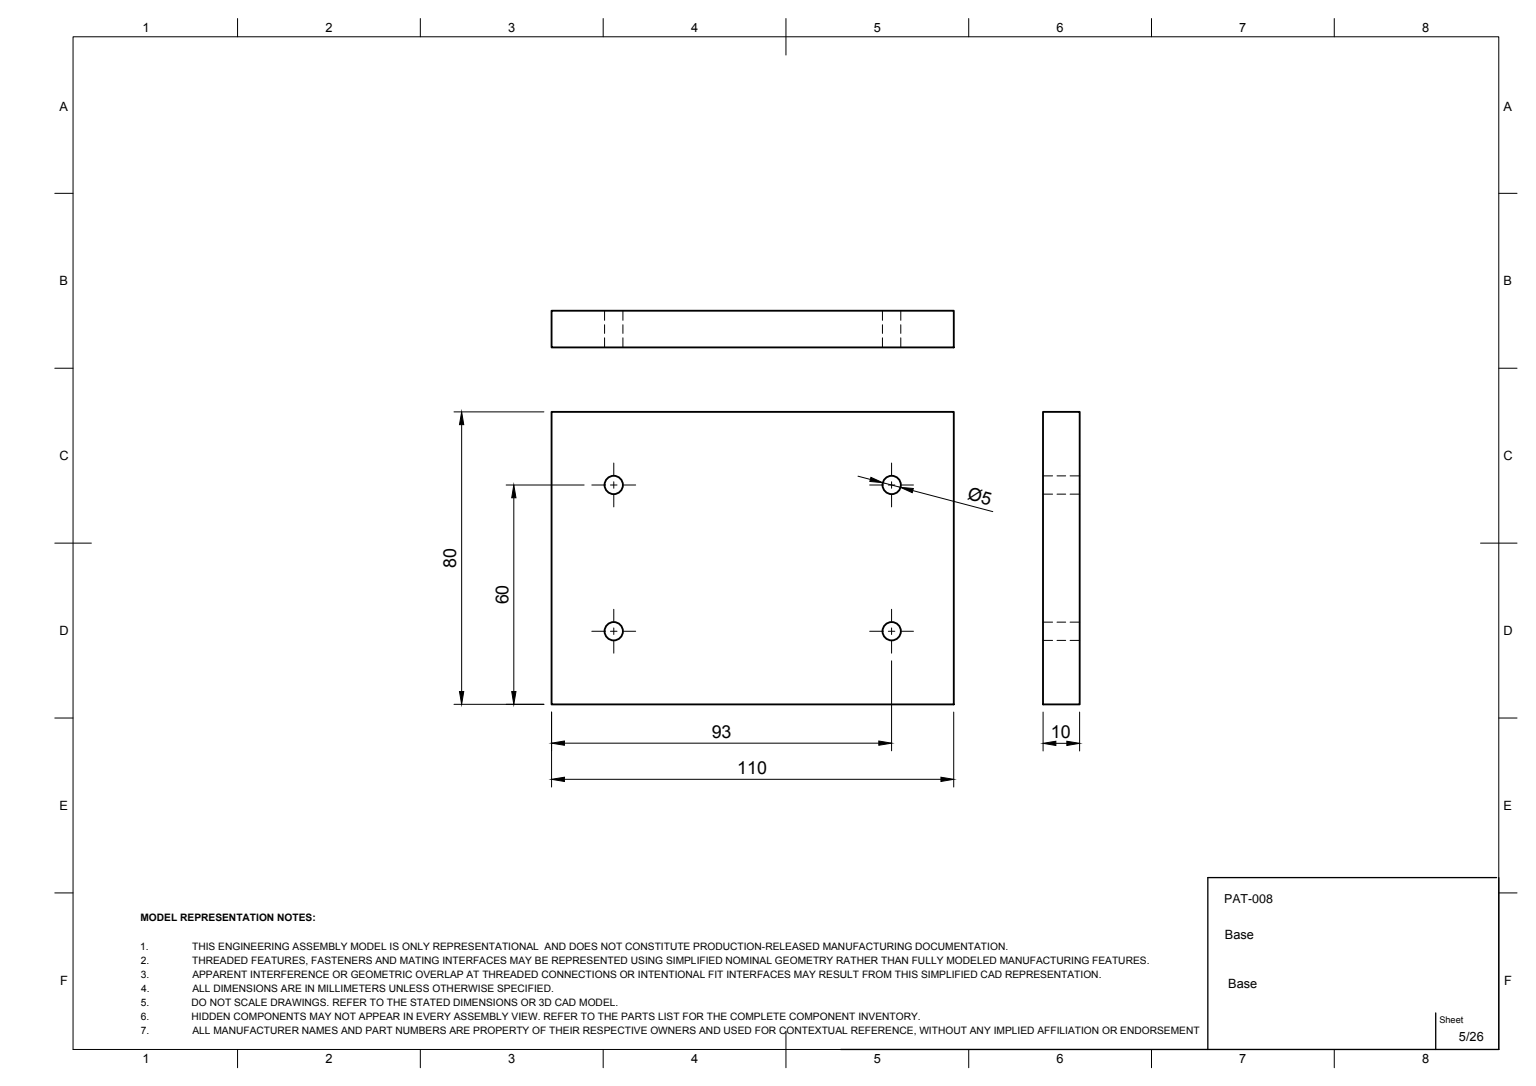
ISO-10303-21;
HEADER;
/* Generated by software containing ST-Developer
 * from STEP Tools, Inc. (www.steptools.com) 
 */

FILE_DESCRIPTION(
/* description */ ('Bearing housing with oil seal and end cap'),
/* implementation_level */ '2;1');

FILE_NAME(
/* name */ 'Base.step',
/* time_stamp */ '2026-10-28T03:23:10-07:00',
/* author */ (''),
/* organization */ (''),
/* preprocessor_version */ 'ST-DEVELOPER v20.2',
/* originating_system */ 'Autodesk Translation Framework v15.17.0.0',
/* authorisation */ '');

FILE_SCHEMA (('AUTOMOTIVE_DESIGN { 1 0 10303 214 3 1 1 }'));
ENDSEC;

DATA;
#10=MECHANICAL_DESIGN_GEOMETRIC_PRESENTATION_REPRESENTATION('',(#259),#7871);
#217=SHAPE_REPRESENTATION_RELATIONSHIP('SRR','None',#7964,#238);
#238=ADVANCED_BREP_SHAPE_REPRESENTATION('',(#288),#7848);
#259=STYLED_ITEM('',(#8132),#288);
#288=MANIFOLD_SOLID_BREP('Body1',#4085);
#315=FACE_BOUND('',#812,.T.);
#316=FACE_BOUND('',#813,.T.);
#317=FACE_BOUND('',#814,.T.);
#318=FACE_BOUND('',#815,.T.);
#319=FACE_BOUND('',#817,.T.);
#320=FACE_BOUND('',#818,.T.);
#321=FACE_BOUND('',#819,.T.);
#322=FACE_BOUND('',#820,.T.);
#408=PLANE('',#4363);
#409=PLANE('',#4364);
#410=PLANE('',#4365);
#411=PLANE('',#4366);
#412=PLANE('',#4367);
#413=PLANE('',#4368);
#552=FACE_OUTER_BOUND('',#803,.T.);
#553=FACE_OUTER_BOUND('',#804,.T.);
#554=FACE_OUTER_BOUND('',#805,.T.);
#555=FACE_OUTER_BOUND('',#806,.T.);
#556=FACE_OUTER_BOUND('',#807,.T.);
#557=FACE_OUTER_BOUND('',#808,.T.);
#558=FACE_OUTER_BOUND('',#809,.T.);
#559=FACE_OUTER_BOUND('',#810,.T.);
#560=FACE_OUTER_BOUND('',#811,.T.);
#561=FACE_OUTER_BOUND('',#816,.T.);
#803=EDGE_LOOP('',(#2743,#2744,#2745,#2746));
#804=EDGE_LOOP('',(#2747,#2748,#2749,#2750));
#805=EDGE_LOOP('',(#2751,#2752,#2753,#2754));
#806=EDGE_LOOP('',(#2755,#2756,#2757,#2758));
#807=EDGE_LOOP('',(#2759,#2760,#2761,#2762));
#808=EDGE_LOOP('',(#2763,#2764,#2765,#2766));
#809=EDGE_LOOP('',(#2767,#2768,#2769,#2770));
#810=EDGE_LOOP('',(#2771,#2772,#2773,#2774));
#811=EDGE_LOOP('',(#2775,#2776,#2777,#2778));
#812=EDGE_LOOP('',(#2779));
#813=EDGE_LOOP('',(#2780));
#814=EDGE_LOOP('',(#2781));
#815=EDGE_LOOP('',(#2782));
#816=EDGE_LOOP('',(#2783,#2784,#2785,#2786));
#817=EDGE_LOOP('',(#2787));
#818=EDGE_LOOP('',(#2788));
#819=EDGE_LOOP('',(#2789));
#820=EDGE_LOOP('',(#2790));
#1147=LINE('',#6213,#1409);
#1148=LINE('',#6219,#1410);
#1149=LINE('',#6225,#1411);
#1150=LINE('',#6231,#1412);
#1151=LINE('',#6236,#1413);
#1152=LINE('',#6238,#1414);
#1153=LINE('',#6240,#1415);
#1154=LINE('',#6241,#1416);
#1155=LINE('',#6244,#1417);
#1156=LINE('',#6246,#1418);
#1157=LINE('',#6247,#1419);
#1158=LINE('',#6250,#1420);
#1159=LINE('',#6252,#1421);
#1160=LINE('',#6253,#1422);
#1161=LINE('',#6255,#1423);
#1162=LINE('',#6256,#1424);
#1409=VECTOR('',#4890,0.25);
#1410=VECTOR('',#4897,0.25);
#1411=VECTOR('',#4904,0.25);
#1412=VECTOR('',#4911,0.25);
#1413=VECTOR('',#4916,1.);
#1414=VECTOR('',#4917,1.);
#1415=VECTOR('',#4918,1.);
#1416=VECTOR('',#4919,1.);
#1417=VECTOR('',#4922,1.);
#1418=VECTOR('',#4923,1.);
#1419=VECTOR('',#4924,1.);
#1420=VECTOR('',#4927,1.);
#1421=VECTOR('',#4928,1.);
#1422=VECTOR('',#4929,1.);
#1423=VECTOR('',#4932,1.);
#1424=VECTOR('',#4933,1.);
#1671=CIRCLE('',#4352,0.25);
#1672=CIRCLE('',#4353,0.25);
#1673=CIRCLE('',#4355,0.25);
#1674=CIRCLE('',#4356,0.25);
#1675=CIRCLE('',#4358,0.25);
#1676=CIRCLE('',#4359,0.25);
#1677=CIRCLE('',#4361,0.25);
#1678=CIRCLE('',#4362,0.25);
#1891=VERTEX_POINT('',#6210);
#1892=VERTEX_POINT('',#6212);
#1893=VERTEX_POINT('',#6216);
#1894=VERTEX_POINT('',#6218);
#1895=VERTEX_POINT('',#6222);
#1896=VERTEX_POINT('',#6224);
#1897=VERTEX_POINT('',#6228);
#1898=VERTEX_POINT('',#6230);
#1899=VERTEX_POINT('',#6234);
#1900=VERTEX_POINT('',#6235);
#1901=VERTEX_POINT('',#6237);
#1902=VERTEX_POINT('',#6239);
#1903=VERTEX_POINT('',#6243);
#1904=VERTEX_POINT('',#6245);
#1905=VERTEX_POINT('',#6249);
#1906=VERTEX_POINT('',#6251);
#2235=EDGE_CURVE('',#1891,#1891,#1671,.T.);
#2236=EDGE_CURVE('',#1891,#1892,#1147,.T.);
#2237=EDGE_CURVE('',#1892,#1892,#1672,.T.);
#2238=EDGE_CURVE('',#1893,#1893,#1673,.T.);
#2239=EDGE_CURVE('',#1893,#1894,#1148,.T.);
#2240=EDGE_CURVE('',#1894,#1894,#1674,.T.);
#2241=EDGE_CURVE('',#1895,#1895,#1675,.T.);
#2242=EDGE_CURVE('',#1895,#1896,#1149,.T.);
#2243=EDGE_CURVE('',#1896,#1896,#1676,.T.);
#2244=EDGE_CURVE('',#1897,#1897,#1677,.T.);
#2245=EDGE_CURVE('',#1897,#1898,#1150,.T.);
#2246=EDGE_CURVE('',#1898,#1898,#1678,.T.);
#2247=EDGE_CURVE('',#1899,#1900,#1151,.T.);
#2248=EDGE_CURVE('',#1900,#1901,#1152,.T.);
#2249=EDGE_CURVE('',#1902,#1901,#1153,.T.);
#2250=EDGE_CURVE('',#1899,#1902,#1154,.T.);
#2251=EDGE_CURVE('',#1903,#1899,#1155,.T.);
#2252=EDGE_CURVE('',#1904,#1902,#1156,.T.);
#2253=EDGE_CURVE('',#1903,#1904,#1157,.T.);
#2254=EDGE_CURVE('',#1905,#1903,#1158,.T.);
#2255=EDGE_CURVE('',#1906,#1904,#1159,.T.);
#2256=EDGE_CURVE('',#1905,#1906,#1160,.T.);
#2257=EDGE_CURVE('',#1900,#1905,#1161,.T.);
#2258=EDGE_CURVE('',#1901,#1906,#1162,.T.);
#2743=ORIENTED_EDGE('',*,*,#2235,.F.);
#2744=ORIENTED_EDGE('',*,*,#2236,.T.);
#2745=ORIENTED_EDGE('',*,*,#2237,.F.);
#2746=ORIENTED_EDGE('',*,*,#2236,.F.);
#2747=ORIENTED_EDGE('',*,*,#2238,.F.);
#2748=ORIENTED_EDGE('',*,*,#2239,.T.);
#2749=ORIENTED_EDGE('',*,*,#2240,.F.);
#2750=ORIENTED_EDGE('',*,*,#2239,.F.);
#2751=ORIENTED_EDGE('',*,*,#2241,.F.);
#2752=ORIENTED_EDGE('',*,*,#2242,.T.);
#2753=ORIENTED_EDGE('',*,*,#2243,.F.);
#2754=ORIENTED_EDGE('',*,*,#2242,.F.);
#2755=ORIENTED_EDGE('',*,*,#2244,.F.);
#2756=ORIENTED_EDGE('',*,*,#2245,.T.);
#2757=ORIENTED_EDGE('',*,*,#2246,.F.);
#2758=ORIENTED_EDGE('',*,*,#2245,.F.);
#2759=ORIENTED_EDGE('',*,*,#2247,.T.);
#2760=ORIENTED_EDGE('',*,*,#2248,.T.);
#2761=ORIENTED_EDGE('',*,*,#2249,.F.);
#2762=ORIENTED_EDGE('',*,*,#2250,.F.);
#2763=ORIENTED_EDGE('',*,*,#2251,.T.);
#2764=ORIENTED_EDGE('',*,*,#2250,.T.);
#2765=ORIENTED_EDGE('',*,*,#2252,.F.);
#2766=ORIENTED_EDGE('',*,*,#2253,.F.);
#2767=ORIENTED_EDGE('',*,*,#2254,.T.);
#2768=ORIENTED_EDGE('',*,*,#2253,.T.);
#2769=ORIENTED_EDGE('',*,*,#2255,.F.);
#2770=ORIENTED_EDGE('',*,*,#2256,.F.);
#2771=ORIENTED_EDGE('',*,*,#2257,.T.);
#2772=ORIENTED_EDGE('',*,*,#2256,.T.);
#2773=ORIENTED_EDGE('',*,*,#2258,.F.);
#2774=ORIENTED_EDGE('',*,*,#2248,.F.);
#2775=ORIENTED_EDGE('',*,*,#2258,.T.);
#2776=ORIENTED_EDGE('',*,*,#2255,.T.);
#2777=ORIENTED_EDGE('',*,*,#2252,.T.);
#2778=ORIENTED_EDGE('',*,*,#2249,.T.);
#2779=ORIENTED_EDGE('',*,*,#2237,.T.);
#2780=ORIENTED_EDGE('',*,*,#2240,.T.);
#2781=ORIENTED_EDGE('',*,*,#2243,.T.);
#2782=ORIENTED_EDGE('',*,*,#2246,.T.);
#2783=ORIENTED_EDGE('',*,*,#2257,.F.);
#2784=ORIENTED_EDGE('',*,*,#2247,.F.);
#2785=ORIENTED_EDGE('',*,*,#2251,.F.);
#2786=ORIENTED_EDGE('',*,*,#2254,.F.);
#2787=ORIENTED_EDGE('',*,*,#2235,.T.);
#2788=ORIENTED_EDGE('',*,*,#2238,.T.);
#2789=ORIENTED_EDGE('',*,*,#2241,.T.);
#2790=ORIENTED_EDGE('',*,*,#2244,.T.);
#3759=CYLINDRICAL_SURFACE('',#4351,0.25);
#3760=CYLINDRICAL_SURFACE('',#4354,0.25);
#3761=CYLINDRICAL_SURFACE('',#4357,0.25);
#3762=CYLINDRICAL_SURFACE('',#4360,0.25);
#3834=ADVANCED_FACE('',(#552),#3759,.F.);
#3835=ADVANCED_FACE('',(#553),#3760,.F.);
#3836=ADVANCED_FACE('',(#554),#3761,.F.);
#3837=ADVANCED_FACE('',(#555),#3762,.F.);
#3838=ADVANCED_FACE('',(#556),#408,.T.);
#3839=ADVANCED_FACE('',(#557),#409,.T.);
#3840=ADVANCED_FACE('',(#558),#410,.T.);
#3841=ADVANCED_FACE('',(#559),#411,.T.);
#3842=ADVANCED_FACE('',(#560,#315,#316,#317,#318),#412,.T.);
#3843=ADVANCED_FACE('',(#561,#319,#320,#321,#322),#413,.F.);
#4085=CLOSED_SHELL('',(#3834,#3835,#3836,#3837,#3838,#3839,#3840,#3841,
#3842,#3843));
#4350=AXIS2_PLACEMENT_3D('',#6208,#4884,#4885);
#4351=AXIS2_PLACEMENT_3D('',#6209,#4886,#4887);
#4352=AXIS2_PLACEMENT_3D('',#6211,#4888,#4889);
#4353=AXIS2_PLACEMENT_3D('',#6214,#4891,#4892);
#4354=AXIS2_PLACEMENT_3D('',#6215,#4893,#4894);
#4355=AXIS2_PLACEMENT_3D('',#6217,#4895,#4896);
#4356=AXIS2_PLACEMENT_3D('',#6220,#4898,#4899);
#4357=AXIS2_PLACEMENT_3D('',#6221,#4900,#4901);
#4358=AXIS2_PLACEMENT_3D('',#6223,#4902,#4903);
#4359=AXIS2_PLACEMENT_3D('',#6226,#4905,#4906);
#4360=AXIS2_PLACEMENT_3D('',#6227,#4907,#4908);
#4361=AXIS2_PLACEMENT_3D('',#6229,#4909,#4910);
#4362=AXIS2_PLACEMENT_3D('',#6232,#4912,#4913);
#4363=AXIS2_PLACEMENT_3D('',#6233,#4914,#4915);
#4364=AXIS2_PLACEMENT_3D('',#6242,#4920,#4921);
#4365=AXIS2_PLACEMENT_3D('',#6248,#4925,#4926);
#4366=AXIS2_PLACEMENT_3D('',#6254,#4930,#4931);
#4367=AXIS2_PLACEMENT_3D('',#6257,#4934,#4935);
#4368=AXIS2_PLACEMENT_3D('',#6258,#4936,#4937);
#4884=DIRECTION('axis',(0.,0.,1.));
#4885=DIRECTION('refdir',(1.,0.,0.));
#4886=DIRECTION('center_axis',(0.,0.,1.));
#4887=DIRECTION('ref_axis',(1.,0.,0.));
#4888=DIRECTION('center_axis',(0.,0.,1.));
#4889=DIRECTION('ref_axis',(1.,0.,0.));
#4890=DIRECTION('',(0.,0.,1.));
#4891=DIRECTION('center_axis',(0.,0.,-1.));
#4892=DIRECTION('ref_axis',(1.,0.,0.));
#4893=DIRECTION('center_axis',(0.,0.,1.));
#4894=DIRECTION('ref_axis',(1.,0.,0.));
#4895=DIRECTION('center_axis',(0.,0.,1.));
#4896=DIRECTION('ref_axis',(1.,0.,0.));
#4897=DIRECTION('',(0.,0.,1.));
#4898=DIRECTION('center_axis',(0.,0.,-1.));
#4899=DIRECTION('ref_axis',(1.,0.,0.));
#4900=DIRECTION('center_axis',(0.,0.,1.));
#4901=DIRECTION('ref_axis',(1.,0.,0.));
#4902=DIRECTION('center_axis',(0.,0.,1.));
#4903=DIRECTION('ref_axis',(1.,0.,0.));
#4904=DIRECTION('',(0.,0.,1.));
#4905=DIRECTION('center_axis',(0.,0.,-1.));
#4906=DIRECTION('ref_axis',(1.,0.,0.));
#4907=DIRECTION('center_axis',(0.,0.,1.));
#4908=DIRECTION('ref_axis',(1.,0.,0.));
#4909=DIRECTION('center_axis',(0.,0.,1.));
#4910=DIRECTION('ref_axis',(1.,0.,0.));
#4911=DIRECTION('',(0.,0.,1.));
#4912=DIRECTION('center_axis',(0.,0.,-1.));
#4913=DIRECTION('ref_axis',(1.,0.,0.));
#4914=DIRECTION('center_axis',(0.,1.,0.));
#4915=DIRECTION('ref_axis',(-1.,0.,0.));
#4916=DIRECTION('',(-1.,0.,0.));
#4917=DIRECTION('',(0.,0.,1.));
#4918=DIRECTION('',(-1.,0.,0.));
#4919=DIRECTION('',(0.,0.,1.));
#4920=DIRECTION('center_axis',(1.,0.,0.));
#4921=DIRECTION('ref_axis',(0.,1.,0.));
#4922=DIRECTION('',(0.,1.,0.));
#4923=DIRECTION('',(0.,1.,0.));
#4924=DIRECTION('',(0.,0.,1.));
#4925=DIRECTION('center_axis',(0.,-1.,0.));
#4926=DIRECTION('ref_axis',(1.,0.,0.));
#4927=DIRECTION('',(1.,0.,0.));
#4928=DIRECTION('',(1.,0.,0.));
#4929=DIRECTION('',(0.,0.,1.));
#4930=DIRECTION('center_axis',(-1.,0.,0.));
#4931=DIRECTION('ref_axis',(0.,-1.,0.));
#4932=DIRECTION('',(0.,-1.,0.));
#4933=DIRECTION('',(0.,-1.,0.));
#4934=DIRECTION('center_axis',(0.,0.,1.));
#4935=DIRECTION('ref_axis',(1.,0.,0.));
#4936=DIRECTION('center_axis',(0.,0.,1.));
#4937=DIRECTION('ref_axis',(1.,0.,0.));
#6208=CARTESIAN_POINT('',(0.,0.,0.));
#6209=CARTESIAN_POINT('Origin',(3.8,1.,-0.1));
#6210=CARTESIAN_POINT('',(3.55,1.,0.));
#6211=CARTESIAN_POINT('Origin',(3.8,1.,0.));
#6212=CARTESIAN_POINT('',(3.55,1.,1.));
#6213=CARTESIAN_POINT('',(3.55,1.,-0.1));
#6214=CARTESIAN_POINT('Origin',(3.8,1.,1.));
#6215=CARTESIAN_POINT('Origin',(-3.8,5.,-0.1));
#6216=CARTESIAN_POINT('',(-4.05,5.,0.));
#6217=CARTESIAN_POINT('Origin',(-3.8,5.,0.));
#6218=CARTESIAN_POINT('',(-4.05,5.,1.));
#6219=CARTESIAN_POINT('',(-4.05,5.,-0.1));
#6220=CARTESIAN_POINT('Origin',(-3.8,5.,1.));
#6221=CARTESIAN_POINT('Origin',(-3.8,1.,-0.1));
#6222=CARTESIAN_POINT('',(-4.05,1.,0.));
#6223=CARTESIAN_POINT('Origin',(-3.8,1.,0.));
#6224=CARTESIAN_POINT('',(-4.05,1.,1.));
#6225=CARTESIAN_POINT('',(-4.05,1.,-0.1));
#6226=CARTESIAN_POINT('Origin',(-3.8,1.,1.));
#6227=CARTESIAN_POINT('Origin',(3.8,5.,-0.1));
#6228=CARTESIAN_POINT('',(3.55,5.,0.));
#6229=CARTESIAN_POINT('Origin',(3.8,5.,0.));
#6230=CARTESIAN_POINT('',(3.55,5.,1.));
#6231=CARTESIAN_POINT('',(3.55,5.,-0.1));
#6232=CARTESIAN_POINT('Origin',(3.8,5.,1.));
#6233=CARTESIAN_POINT('Origin',(5.5,7.,0.));
#6234=CARTESIAN_POINT('',(5.5,7.,0.));
#6235=CARTESIAN_POINT('',(-5.5,7.,0.));
#6236=CARTESIAN_POINT('',(5.5,7.,0.));
#6237=CARTESIAN_POINT('',(-5.5,7.,1.));
#6238=CARTESIAN_POINT('',(-5.5,7.,0.));
#6239=CARTESIAN_POINT('',(5.5,7.,1.));
#6240=CARTESIAN_POINT('',(5.5,7.,1.));
#6241=CARTESIAN_POINT('',(5.5,7.,0.));
#6242=CARTESIAN_POINT('Origin',(5.5,-1.,0.));
#6243=CARTESIAN_POINT('',(5.5,-1.,0.));
#6244=CARTESIAN_POINT('',(5.5,-1.,0.));
#6245=CARTESIAN_POINT('',(5.5,-1.,1.));
#6246=CARTESIAN_POINT('',(5.5,-1.,1.));
#6247=CARTESIAN_POINT('',(5.5,-1.,0.));
#6248=CARTESIAN_POINT('Origin',(-5.5,-1.,0.));
#6249=CARTESIAN_POINT('',(-5.5,-1.,0.));
#6250=CARTESIAN_POINT('',(-5.5,-1.,0.));
#6251=CARTESIAN_POINT('',(-5.5,-1.,1.));
#6252=CARTESIAN_POINT('',(-5.5,-1.,1.));
#6253=CARTESIAN_POINT('',(-5.5,-1.,0.));
#6254=CARTESIAN_POINT('Origin',(-5.5,7.,0.));
#6255=CARTESIAN_POINT('',(-5.5,7.,0.));
#6256=CARTESIAN_POINT('',(-5.5,7.,1.));
#6257=CARTESIAN_POINT('Origin',(0.,3.,1.));
#6258=CARTESIAN_POINT('Origin',(0.,3.,0.));
#7822=UNCERTAINTY_MEASURE_WITH_UNIT(LENGTH_MEASURE(0.001),#7872,
'DISTANCE_ACCURACY_VALUE',
'Maximum model space distance between geometric entities at asserted c
onnectivities');
#7845=UNCERTAINTY_MEASURE_WITH_UNIT(LENGTH_MEASURE(0.001),#7872,
'DISTANCE_ACCURACY_VALUE',
'Maximum model space distance between geometric entities at asserted c
onnectivities');
#7848=(
GEOMETRIC_REPRESENTATION_CONTEXT(3)
GLOBAL_UNCERTAINTY_ASSIGNED_CONTEXT((#7822))
GLOBAL_UNIT_ASSIGNED_CONTEXT((#7872,#7874,#7875))
REPRESENTATION_CONTEXT('','3D')
);
#7871=(
GEOMETRIC_REPRESENTATION_CONTEXT(3)
GLOBAL_UNCERTAINTY_ASSIGNED_CONTEXT((#7845))
GLOBAL_UNIT_ASSIGNED_CONTEXT((#7872,#7874,#7875))
REPRESENTATION_CONTEXT('','3D')
);
#7872=(
LENGTH_UNIT()
NAMED_UNIT(*)
SI_UNIT(.CENTI.,.METRE.)
);
#7874=(
NAMED_UNIT(*)
PLANE_ANGLE_UNIT()
SI_UNIT($,.RADIAN.)
);
#7875=(
NAMED_UNIT(*)
SI_UNIT($,.STERADIAN.)
SOLID_ANGLE_UNIT()
);
#7878=SHAPE_DEFINITION_REPRESENTATION(#7903,#7964);
#7903=PRODUCT_DEFINITION_SHAPE('',$,#7990);
#7964=SHAPE_REPRESENTATION('',(#4350),#7848);
#7987=PRODUCT_DEFINITION_CONTEXT('part definition',#8064,'design');
#7990=PRODUCT_DEFINITION('Base','Base',#8015,#7987);
#8015=PRODUCT_DEFINITION_FORMATION('',$,#8068);
#8064=APPLICATION_CONTEXT(
'Core Data for Automotive Mechanical Design Process');
#8065=PRODUCT_CONTEXT('part definition',#8064,'mechanical');
#8068=PRODUCT('Base','Base','Base',(#8065));
#8126=COLOUR_RGB('Dark Blue',0.08,0.2,0.34);
#8127=FILL_AREA_STYLE_COLOUR('',#8126);
#8128=FILL_AREA_STYLE('',(#8127));
#8129=SURFACE_STYLE_FILL_AREA(#8128);
#8130=SURFACE_SIDE_STYLE('',(#8129));
#8131=SURFACE_STYLE_USAGE(.BOTH.,#8130);
#8132=PRESENTATION_STYLE_ASSIGNMENT((#8131));
ENDSEC;
END-ISO-10303-21;
